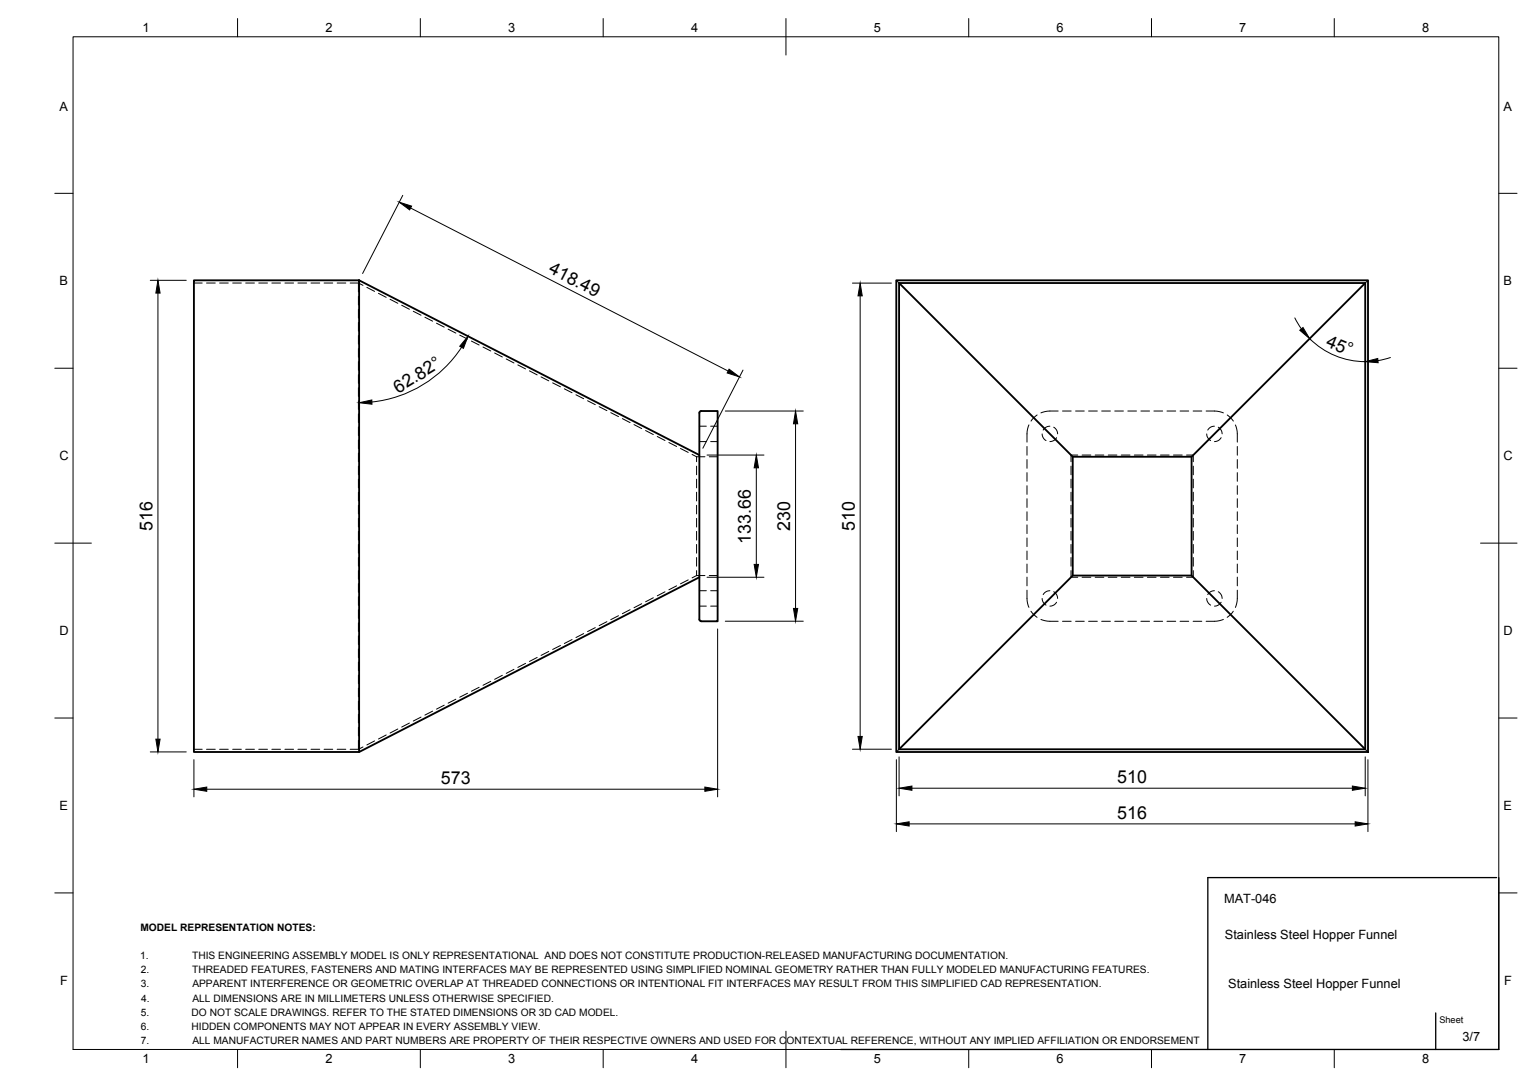
ISO-10303-21;
HEADER;
/* Generated by software containing ST-Developer
 * from STEP Tools, Inc. (www.steptools.com) 
 */

FILE_DESCRIPTION(
/* description */ ('STEP AP214'),
/* implementation_level */ '2;1');

FILE_NAME(
/* name */ 'Stainless Steel Hopper Funnel.step',
/* time_stamp */ '2026-11-14T22:16:48-08:00',
/* author */ (''),
/* organization */ (''),
/* preprocessor_version */ 'ST-DEVELOPER v20.2',
/* originating_system */ 'Autodesk Translation Framework v15.17.0.0',
/* authorisation */ '');

FILE_SCHEMA (('AUTOMOTIVE_DESIGN { 1 0 10303 214 3 1 1 }'));
ENDSEC;

DATA;
#10=MECHANICAL_DESIGN_GEOMETRIC_PRESENTATION_REPRESENTATION('',(#5472),#276462);
#5460=SHAPE_REPRESENTATION_RELATIONSHIP('SRR','None',#276488,#5466);
#5466=ADVANCED_BREP_SHAPE_REPRESENTATION('',(#5501),#276456);
#5472=STYLED_ITEM('',(#276527),#5501);
#5501=MANIFOLD_SOLID_BREP('Body1',#98697);
#5529=TOROIDAL_SURFACE('',#98859,23.,2.);
#5530=TOROIDAL_SURFACE('',#98866,23.,2.);
#5531=TOROIDAL_SURFACE('',#98868,23.,2.);
#5532=TOROIDAL_SURFACE('',#98874,23.,2.);
#6322=FACE_BOUND('',#13733,.T.);
#6323=FACE_BOUND('',#13751,.T.);
#6324=FACE_BOUND('',#13752,.T.);
#6325=FACE_BOUND('',#13753,.T.);
#6326=FACE_BOUND('',#13754,.T.);
#6327=FACE_BOUND('',#13755,.T.);
#6328=FACE_BOUND('',#13757,.T.);
#6329=FACE_BOUND('',#13758,.T.);
#6330=FACE_BOUND('',#13759,.T.);
#6331=FACE_BOUND('',#13760,.T.);
#6332=FACE_BOUND('',#13761,.T.);
#6446=PLANE('',#98816);
#6447=PLANE('',#98817);
#6448=PLANE('',#98818);
#6449=PLANE('',#98819);
#6450=PLANE('',#98820);
#6451=PLANE('',#98821);
#6452=PLANE('',#98822);
#6453=PLANE('',#98823);
#6454=PLANE('',#98824);
#6455=PLANE('',#98825);
#6456=PLANE('',#98826);
#6457=PLANE('',#98827);
#6458=PLANE('',#98828);
#6459=PLANE('',#98829);
#6460=PLANE('',#98830);
#6461=PLANE('',#98831);
#6462=PLANE('',#98832);
#6463=PLANE('',#98833);
#6464=PLANE('',#98834);
#6465=PLANE('',#98835);
#6466=PLANE('',#98836);
#6467=PLANE('',#98837);
#6468=PLANE('',#98842);
#6469=PLANE('',#98847);
#6470=PLANE('',#98848);
#6471=PLANE('',#98849);
#6472=PLANE('',#98850);
#7614=FACE_OUTER_BOUND('',#13724,.T.);
#7615=FACE_OUTER_BOUND('',#13725,.T.);
#7616=FACE_OUTER_BOUND('',#13726,.T.);
#7617=FACE_OUTER_BOUND('',#13727,.T.);
#7618=FACE_OUTER_BOUND('',#13728,.T.);
#7619=FACE_OUTER_BOUND('',#13729,.T.);
#7620=FACE_OUTER_BOUND('',#13730,.T.);
#7621=FACE_OUTER_BOUND('',#13731,.T.);
#7622=FACE_OUTER_BOUND('',#13732,.T.);
#7623=FACE_OUTER_BOUND('',#13734,.T.);
#7624=FACE_OUTER_BOUND('',#13735,.T.);
#7625=FACE_OUTER_BOUND('',#13736,.T.);
#7626=FACE_OUTER_BOUND('',#13737,.T.);
#7627=FACE_OUTER_BOUND('',#13738,.T.);
#7628=FACE_OUTER_BOUND('',#13739,.T.);
#7629=FACE_OUTER_BOUND('',#13740,.T.);
#7630=FACE_OUTER_BOUND('',#13741,.T.);
#7631=FACE_OUTER_BOUND('',#13742,.T.);
#7632=FACE_OUTER_BOUND('',#13743,.T.);
#7633=FACE_OUTER_BOUND('',#13744,.T.);
#7634=FACE_OUTER_BOUND('',#13745,.T.);
#7635=FACE_OUTER_BOUND('',#13746,.T.);
#7636=FACE_OUTER_BOUND('',#13747,.T.);
#7637=FACE_OUTER_BOUND('',#13748,.T.);
#7638=FACE_OUTER_BOUND('',#13749,.T.);
#7639=FACE_OUTER_BOUND('',#13750,.T.);
#7640=FACE_OUTER_BOUND('',#13756,.T.);
#7641=FACE_OUTER_BOUND('',#13762,.T.);
#7642=FACE_OUTER_BOUND('',#13763,.T.);
#7643=FACE_OUTER_BOUND('',#13764,.T.);
#7644=FACE_OUTER_BOUND('',#13765,.T.);
#7645=FACE_OUTER_BOUND('',#13766,.T.);
#7646=FACE_OUTER_BOUND('',#13767,.T.);
#7647=FACE_OUTER_BOUND('',#13768,.T.);
#7648=FACE_OUTER_BOUND('',#13769,.T.);
#7649=FACE_OUTER_BOUND('',#13770,.T.);
#7650=FACE_OUTER_BOUND('',#13771,.T.);
#7651=FACE_OUTER_BOUND('',#13772,.T.);
#7652=FACE_OUTER_BOUND('',#13773,.T.);
#7653=FACE_OUTER_BOUND('',#13774,.T.);
#7654=FACE_OUTER_BOUND('',#13775,.T.);
#7655=FACE_OUTER_BOUND('',#13776,.T.);
#7656=FACE_OUTER_BOUND('',#13777,.T.);
#13724=EDGE_LOOP('',(#60425,#60426,#60427,#60428));
#13725=EDGE_LOOP('',(#60429,#60430,#60431,#60432));
#13726=EDGE_LOOP('',(#60433,#60434,#60435,#60436));
#13727=EDGE_LOOP('',(#60437,#60438,#60439,#60440));
#13728=EDGE_LOOP('',(#60441,#60442,#60443,#60444));
#13729=EDGE_LOOP('',(#60445,#60446,#60447,#60448));
#13730=EDGE_LOOP('',(#60449,#60450,#60451,#60452));
#13731=EDGE_LOOP('',(#60453,#60454,#60455,#60456));
#13732=EDGE_LOOP('',(#60457,#60458,#60459,#60460));
#13733=EDGE_LOOP('',(#60461,#60462,#60463,#60464));
#13734=EDGE_LOOP('',(#60465,#60466,#60467,#60468));
#13735=EDGE_LOOP('',(#60469,#60470,#60471,#60472));
#13736=EDGE_LOOP('',(#60473,#60474,#60475,#60476));
#13737=EDGE_LOOP('',(#60477,#60478,#60479,#60480));
#13738=EDGE_LOOP('',(#60481,#60482,#60483,#60484));
#13739=EDGE_LOOP('',(#60485,#60486,#60487,#60488));
#13740=EDGE_LOOP('',(#60489,#60490,#60491,#60492));
#13741=EDGE_LOOP('',(#60493,#60494,#60495,#60496));
#13742=EDGE_LOOP('',(#60497,#60498,#60499,#60500));
#13743=EDGE_LOOP('',(#60501,#60502,#60503,#60504));
#13744=EDGE_LOOP('',(#60505,#60506,#60507,#60508));
#13745=EDGE_LOOP('',(#60509,#60510,#60511,#60512));
#13746=EDGE_LOOP('',(#60513,#60514,#60515,#60516));
#13747=EDGE_LOOP('',(#60517,#60518,#60519,#60520));
#13748=EDGE_LOOP('',(#60521,#60522,#60523,#60524));
#13749=EDGE_LOOP('',(#60525,#60526,#60527,#60528));
#13750=EDGE_LOOP('',(#60529,#60530,#60531,#60532,#60533,#60534,#60535,#60536));
#13751=EDGE_LOOP('',(#60537));
#13752=EDGE_LOOP('',(#60538));
#13753=EDGE_LOOP('',(#60539));
#13754=EDGE_LOOP('',(#60540));
#13755=EDGE_LOOP('',(#60541,#60542,#60543,#60544));
#13756=EDGE_LOOP('',(#60545,#60546,#60547,#60548,#60549,#60550,#60551,#60552));
#13757=EDGE_LOOP('',(#60553,#60554,#60555,#60556));
#13758=EDGE_LOOP('',(#60557));
#13759=EDGE_LOOP('',(#60558));
#13760=EDGE_LOOP('',(#60559));
#13761=EDGE_LOOP('',(#60560));
#13762=EDGE_LOOP('',(#60561,#60562,#60563,#60564));
#13763=EDGE_LOOP('',(#60565,#60566,#60567,#60568));
#13764=EDGE_LOOP('',(#60569,#60570,#60571,#60572));
#13765=EDGE_LOOP('',(#60573,#60574,#60575,#60576));
#13766=EDGE_LOOP('',(#60577,#60578,#60579,#60580));
#13767=EDGE_LOOP('',(#60581,#60582,#60583,#60584));
#13768=EDGE_LOOP('',(#60585,#60586,#60587,#60588));
#13769=EDGE_LOOP('',(#60589,#60590,#60591,#60592));
#13770=EDGE_LOOP('',(#60593,#60594,#60595,#60596));
#13771=EDGE_LOOP('',(#60597,#60598,#60599,#60600));
#13772=EDGE_LOOP('',(#60601,#60602,#60603,#60604));
#13773=EDGE_LOOP('',(#60605,#60606,#60607,#60608));
#13774=EDGE_LOOP('',(#60609,#60610,#60611,#60612));
#13775=EDGE_LOOP('',(#60613,#60614,#60615,#60616));
#13776=EDGE_LOOP('',(#60617,#60618,#60619,#60620));
#13777=EDGE_LOOP('',(#60621,#60622,#60623,#60624));
#19958=LINE('',#142648,#25185);
#19959=LINE('',#142654,#25186);
#19960=LINE('',#142660,#25187);
#19961=LINE('',#142666,#25188);
#19962=LINE('',#142671,#25189);
#19963=LINE('',#142673,#25190);
#19964=LINE('',#142675,#25191);
#19965=LINE('',#142676,#25192);
#19966=LINE('',#142679,#25193);
#19967=LINE('',#142681,#25194);
#19968=LINE('',#142682,#25195);
#19969=LINE('',#142685,#25196);
#19970=LINE('',#142687,#25197);
#19971=LINE('',#142688,#25198);
#19972=LINE('',#142690,#25199);
#19973=LINE('',#142691,#25200);
#19974=LINE('',#142695,#25201);
#19975=LINE('',#142697,#25202);
#19976=LINE('',#142699,#25203);
#19977=LINE('',#142700,#25204);
#19978=LINE('',#142703,#25205);
#19979=LINE('',#142705,#25206);
#19980=LINE('',#142706,#25207);
#19981=LINE('',#142709,#25208);
#19982=LINE('',#142710,#25209);
#19983=LINE('',#142713,#25210);
#19984=LINE('',#142714,#25211);
#19985=LINE('',#142716,#25212);
#19986=LINE('',#142719,#25213);
#19987=LINE('',#142721,#25214);
#19988=LINE('',#142722,#25215);
#19989=LINE('',#142725,#25216);
#19990=LINE('',#142726,#25217);
#19991=LINE('',#142729,#25218);
#19992=LINE('',#142730,#25219);
#19993=LINE('',#142732,#25220);
#19994=LINE('',#142735,#25221);
#19995=LINE('',#142737,#25222);
#19996=LINE('',#142738,#25223);
#19997=LINE('',#142741,#25224);
#19998=LINE('',#142742,#25225);
#19999=LINE('',#142745,#25226);
#20000=LINE('',#142746,#25227);
#20001=LINE('',#142748,#25228);
#20002=LINE('',#142751,#25229);
#20003=LINE('',#142753,#25230);
#20004=LINE('',#142754,#25231);
#20005=LINE('',#142757,#25232);
#20006=LINE('',#142758,#25233);
#20007=LINE('',#142761,#25234);
#20008=LINE('',#142762,#25235);
#20009=LINE('',#142764,#25236);
#20010=LINE('',#142768,#25237);
#20011=LINE('',#142772,#25238);
#20012=LINE('',#142776,#25239);
#20013=LINE('',#142780,#25240);
#20014=LINE('',#142785,#25241);
#20015=LINE('',#142789,#25242);
#20016=LINE('',#142793,#25243);
#20017=LINE('',#142797,#25244);
#20018=LINE('',#142801,#25245);
#20019=LINE('',#142803,#25246);
#20020=LINE('',#142804,#25247);
#20021=LINE('',#142807,#25248);
#20022=LINE('',#142809,#25249);
#20023=LINE('',#142810,#25250);
#20024=LINE('',#142813,#25251);
#20025=LINE('',#142815,#25252);
#20026=LINE('',#142816,#25253);
#20027=LINE('',#142819,#25254);
#20028=LINE('',#142821,#25255);
#20029=LINE('',#142822,#25256);
#25185=VECTOR('',#111681,8.4455);
#25186=VECTOR('',#111688,8.4455);
#25187=VECTOR('',#111695,8.4455);
#25188=VECTOR('',#111702,8.4455);
#25189=VECTOR('',#111707,1000.);
#25190=VECTOR('',#111708,1000.);
#25191=VECTOR('',#111709,1000.);
#25192=VECTOR('',#111710,1000.);
#25193=VECTOR('',#111713,1000.);
#25194=VECTOR('',#111714,1000.);
#25195=VECTOR('',#111715,1000.);
#25196=VECTOR('',#111718,1000.);
#25197=VECTOR('',#111719,1000.);
#25198=VECTOR('',#111720,1000.);
#25199=VECTOR('',#111723,1000.);
#25200=VECTOR('',#111724,1000.);
#25201=VECTOR('',#111727,1000.);
#25202=VECTOR('',#111728,1000.);
#25203=VECTOR('',#111729,1000.);
#25204=VECTOR('',#111730,1000.);
#25205=VECTOR('',#111733,1000.);
#25206=VECTOR('',#111734,1000.);
#25207=VECTOR('',#111735,1000.);
#25208=VECTOR('',#111738,1000.);
#25209=VECTOR('',#111739,1000.);
#25210=VECTOR('',#111742,1000.);
#25211=VECTOR('',#111743,1000.);
#25212=VECTOR('',#111746,1000.);
#25213=VECTOR('',#111749,1000.);
#25214=VECTOR('',#111750,1000.);
#25215=VECTOR('',#111751,1000.);
#25216=VECTOR('',#111754,1000.);
#25217=VECTOR('',#111755,1000.);
#25218=VECTOR('',#111758,1000.);
#25219=VECTOR('',#111759,1000.);
#25220=VECTOR('',#111762,1000.);
#25221=VECTOR('',#111765,1000.);
#25222=VECTOR('',#111766,1000.);
#25223=VECTOR('',#111767,1000.);
#25224=VECTOR('',#111770,1000.);
#25225=VECTOR('',#111771,1000.);
#25226=VECTOR('',#111774,1000.);
#25227=VECTOR('',#111775,1000.);
#25228=VECTOR('',#111778,1000.);
#25229=VECTOR('',#111781,1000.);
#25230=VECTOR('',#111782,1000.);
#25231=VECTOR('',#111783,1000.);
#25232=VECTOR('',#111786,1000.);
#25233=VECTOR('',#111787,1000.);
#25234=VECTOR('',#111790,1000.);
#25235=VECTOR('',#111791,1000.);
#25236=VECTOR('',#111794,1000.);
#25237=VECTOR('',#111797,1000.);
#25238=VECTOR('',#111800,1000.);
#25239=VECTOR('',#111803,1000.);
#25240=VECTOR('',#111806,1000.);
#25241=VECTOR('',#111811,1000.);
#25242=VECTOR('',#111814,1000.);
#25243=VECTOR('',#111817,1000.);
#25244=VECTOR('',#111820,1000.);
#25245=VECTOR('',#111825,1000.);
#25246=VECTOR('',#111826,1000.);
#25247=VECTOR('',#111827,1000.);
#25248=VECTOR('',#111830,1000.);
#25249=VECTOR('',#111831,1000.);
#25250=VECTOR('',#111832,1000.);
#25251=VECTOR('',#111835,1000.);
#25252=VECTOR('',#111836,1000.);
#25253=VECTOR('',#111837,1000.);
#25254=VECTOR('',#111840,1000.);
#25255=VECTOR('',#111841,1000.);
#25256=VECTOR('',#111842,1000.);
#30412=CIRCLE('',#98805,8.4455);
#30413=CIRCLE('',#98806,8.4455);
#30414=CIRCLE('',#98808,8.4455);
#30415=CIRCLE('',#98809,8.4455);
#30416=CIRCLE('',#98811,8.4455);
#30417=CIRCLE('',#98812,8.4455);
#30418=CIRCLE('',#98814,8.4455);
#30419=CIRCLE('',#98815,8.4455);
#30420=CIRCLE('',#98838,23.);
#30421=CIRCLE('',#98839,23.);
#30422=CIRCLE('',#98840,23.);
#30423=CIRCLE('',#98841,23.);
#30424=CIRCLE('',#98843,25.);
#30425=CIRCLE('',#98844,25.);
#30426=CIRCLE('',#98845,25.);
#30427=CIRCLE('',#98846,25.);
#30428=CIRCLE('',#98852,25.);
#30429=CIRCLE('',#98854,25.);
#30430=CIRCLE('',#98856,25.);
#30431=CIRCLE('',#98858,25.);
#30432=CIRCLE('',#98860,2.);
#30433=CIRCLE('',#98861,2.);
#30434=CIRCLE('',#98863,2.);
#30435=CIRCLE('',#98865,2.);
#30436=CIRCLE('',#98867,2.);
#30437=CIRCLE('',#98869,2.);
#30438=CIRCLE('',#98871,2.);
#30439=CIRCLE('',#98873,2.);
#36559=VERTEX_POINT('',#142645);
#36560=VERTEX_POINT('',#142647);
#36561=VERTEX_POINT('',#142651);
#36562=VERTEX_POINT('',#142653);
#36563=VERTEX_POINT('',#142657);
#36564=VERTEX_POINT('',#142659);
#36565=VERTEX_POINT('',#142663);
#36566=VERTEX_POINT('',#142665);
#36567=VERTEX_POINT('',#142669);
#36568=VERTEX_POINT('',#142670);
#36569=VERTEX_POINT('',#142672);
#36570=VERTEX_POINT('',#142674);
#36571=VERTEX_POINT('',#142678);
#36572=VERTEX_POINT('',#142680);
#36573=VERTEX_POINT('',#142684);
#36574=VERTEX_POINT('',#142686);
#36575=VERTEX_POINT('',#142693);
#36576=VERTEX_POINT('',#142694);
#36577=VERTEX_POINT('',#142696);
#36578=VERTEX_POINT('',#142698);
#36579=VERTEX_POINT('',#142702);
#36580=VERTEX_POINT('',#142704);
#36581=VERTEX_POINT('',#142708);
#36582=VERTEX_POINT('',#142712);
#36583=VERTEX_POINT('',#142718);
#36584=VERTEX_POINT('',#142720);
#36585=VERTEX_POINT('',#142724);
#36586=VERTEX_POINT('',#142728);
#36587=VERTEX_POINT('',#142734);
#36588=VERTEX_POINT('',#142736);
#36589=VERTEX_POINT('',#142740);
#36590=VERTEX_POINT('',#142744);
#36591=VERTEX_POINT('',#142750);
#36592=VERTEX_POINT('',#142752);
#36593=VERTEX_POINT('',#142756);
#36594=VERTEX_POINT('',#142760);
#36595=VERTEX_POINT('',#142766);
#36596=VERTEX_POINT('',#142767);
#36597=VERTEX_POINT('',#142769);
#36598=VERTEX_POINT('',#142771);
#36599=VERTEX_POINT('',#142773);
#36600=VERTEX_POINT('',#142775);
#36601=VERTEX_POINT('',#142777);
#36602=VERTEX_POINT('',#142779);
#36603=VERTEX_POINT('',#142783);
#36604=VERTEX_POINT('',#142784);
#36605=VERTEX_POINT('',#142786);
#36606=VERTEX_POINT('',#142788);
#36607=VERTEX_POINT('',#142790);
#36608=VERTEX_POINT('',#142792);
#36609=VERTEX_POINT('',#142794);
#36610=VERTEX_POINT('',#142796);
#36611=VERTEX_POINT('',#142800);
#36612=VERTEX_POINT('',#142802);
#36613=VERTEX_POINT('',#142806);
#36614=VERTEX_POINT('',#142808);
#36615=VERTEX_POINT('',#142812);
#36616=VERTEX_POINT('',#142814);
#36617=VERTEX_POINT('',#142818);
#36618=VERTEX_POINT('',#142820);
#45491=EDGE_CURVE('',#36559,#36559,#30412,.T.);
#45492=EDGE_CURVE('',#36559,#36560,#19958,.T.);
#45493=EDGE_CURVE('',#36560,#36560,#30413,.T.);
#45494=EDGE_CURVE('',#36561,#36561,#30414,.T.);
#45495=EDGE_CURVE('',#36561,#36562,#19959,.T.);
#45496=EDGE_CURVE('',#36562,#36562,#30415,.T.);
#45497=EDGE_CURVE('',#36563,#36563,#30416,.T.);
#45498=EDGE_CURVE('',#36563,#36564,#19960,.T.);
#45499=EDGE_CURVE('',#36564,#36564,#30417,.T.);
#45500=EDGE_CURVE('',#36565,#36565,#30418,.T.);
#45501=EDGE_CURVE('',#36565,#36566,#19961,.T.);
#45502=EDGE_CURVE('',#36566,#36566,#30419,.T.);
#45503=EDGE_CURVE('',#36567,#36568,#19962,.T.);
#45504=EDGE_CURVE('',#36569,#36567,#19963,.T.);
#45505=EDGE_CURVE('',#36569,#36570,#19964,.T.);
#45506=EDGE_CURVE('',#36570,#36568,#19965,.T.);
#45507=EDGE_CURVE('',#36571,#36567,#19966,.T.);
#45508=EDGE_CURVE('',#36572,#36571,#19967,.T.);
#45509=EDGE_CURVE('',#36572,#36569,#19968,.T.);
#45510=EDGE_CURVE('',#36573,#36571,#19969,.T.);
#45511=EDGE_CURVE('',#36574,#36573,#19970,.T.);
#45512=EDGE_CURVE('',#36574,#36572,#19971,.T.);
#45513=EDGE_CURVE('',#36568,#36573,#19972,.T.);
#45514=EDGE_CURVE('',#36570,#36574,#19973,.T.);
#45515=EDGE_CURVE('',#36575,#36576,#19974,.T.);
#45516=EDGE_CURVE('',#36577,#36575,#19975,.T.);
#45517=EDGE_CURVE('',#36578,#36577,#19976,.T.);
#45518=EDGE_CURVE('',#36576,#36578,#19977,.T.);
#45519=EDGE_CURVE('',#36579,#36574,#19978,.T.);
#45520=EDGE_CURVE('',#36580,#36570,#19979,.T.);
#45521=EDGE_CURVE('',#36579,#36580,#19980,.T.);
#45522=EDGE_CURVE('',#36581,#36569,#19981,.T.);
#45523=EDGE_CURVE('',#36580,#36581,#19982,.T.);
#45524=EDGE_CURVE('',#36582,#36572,#19983,.T.);
#45525=EDGE_CURVE('',#36582,#36579,#19984,.T.);
#45526=EDGE_CURVE('',#36581,#36582,#19985,.T.);
#45527=EDGE_CURVE('',#36583,#36576,#19986,.T.);
#45528=EDGE_CURVE('',#36584,#36583,#19987,.T.);
#45529=EDGE_CURVE('',#36584,#36575,#19988,.T.);
#45530=EDGE_CURVE('',#36585,#36584,#19989,.T.);
#45531=EDGE_CURVE('',#36585,#36577,#19990,.T.);
#45532=EDGE_CURVE('',#36586,#36585,#19991,.T.);
#45533=EDGE_CURVE('',#36586,#36578,#19992,.T.);
#45534=EDGE_CURVE('',#36583,#36586,#19993,.T.);
#45535=EDGE_CURVE('',#36587,#36586,#19994,.T.);
#45536=EDGE_CURVE('',#36587,#36588,#19995,.T.);
#45537=EDGE_CURVE('',#36588,#36583,#19996,.T.);
#45538=EDGE_CURVE('',#36588,#36589,#19997,.T.);
#45539=EDGE_CURVE('',#36589,#36584,#19998,.T.);
#45540=EDGE_CURVE('',#36590,#36585,#19999,.T.);
#45541=EDGE_CURVE('',#36590,#36587,#20000,.T.);
#45542=EDGE_CURVE('',#36589,#36590,#20001,.T.);
#45543=EDGE_CURVE('',#36591,#36587,#20002,.T.);
#45544=EDGE_CURVE('',#36591,#36592,#20003,.T.);
#45545=EDGE_CURVE('',#36592,#36588,#20004,.T.);
#45546=EDGE_CURVE('',#36592,#36593,#20005,.T.);
#45547=EDGE_CURVE('',#36593,#36589,#20006,.T.);
#45548=EDGE_CURVE('',#36593,#36594,#20007,.T.);
#45549=EDGE_CURVE('',#36594,#36590,#20008,.T.);
#45550=EDGE_CURVE('',#36594,#36591,#20009,.T.);
#45551=EDGE_CURVE('',#36595,#36596,#20010,.T.);
#45552=EDGE_CURVE('',#36596,#36597,#30420,.T.);
#45553=EDGE_CURVE('',#36597,#36598,#20011,.T.);
#45554=EDGE_CURVE('',#36598,#36599,#30421,.T.);
#45555=EDGE_CURVE('',#36599,#36600,#20012,.T.);
#45556=EDGE_CURVE('',#36600,#36601,#30422,.T.);
#45557=EDGE_CURVE('',#36601,#36602,#20013,.T.);
#45558=EDGE_CURVE('',#36602,#36595,#30423,.T.);
#45559=EDGE_CURVE('',#36603,#36604,#20014,.T.);
#45560=EDGE_CURVE('',#36604,#36605,#30424,.T.);
#45561=EDGE_CURVE('',#36605,#36606,#20015,.T.);
#45562=EDGE_CURVE('',#36606,#36607,#30425,.T.);
#45563=EDGE_CURVE('',#36607,#36608,#20016,.T.);
#45564=EDGE_CURVE('',#36608,#36609,#30426,.T.);
#45565=EDGE_CURVE('',#36609,#36610,#20017,.T.);
#45566=EDGE_CURVE('',#36610,#36603,#30427,.T.);
#45567=EDGE_CURVE('',#36603,#36611,#20018,.T.);
#45568=EDGE_CURVE('',#36611,#36612,#20019,.T.);
#45569=EDGE_CURVE('',#36612,#36604,#20020,.T.);
#45570=EDGE_CURVE('',#36605,#36613,#20021,.T.);
#45571=EDGE_CURVE('',#36613,#36614,#20022,.T.);
#45572=EDGE_CURVE('',#36614,#36606,#20023,.T.);
#45573=EDGE_CURVE('',#36607,#36615,#20024,.T.);
#45574=EDGE_CURVE('',#36615,#36616,#20025,.T.);
#45575=EDGE_CURVE('',#36616,#36608,#20026,.T.);
#45576=EDGE_CURVE('',#36609,#36617,#20027,.T.);
#45577=EDGE_CURVE('',#36617,#36618,#20028,.T.);
#45578=EDGE_CURVE('',#36618,#36610,#20029,.T.);
#45579=EDGE_CURVE('',#36612,#36613,#30428,.T.);
#45580=EDGE_CURVE('',#36618,#36611,#30429,.T.);
#45581=EDGE_CURVE('',#36616,#36617,#30430,.T.);
#45582=EDGE_CURVE('',#36614,#36615,#30431,.T.);
#45583=EDGE_CURVE('',#36615,#36600,#30432,.T.);
#45584=EDGE_CURVE('',#36601,#36614,#30433,.T.);
#45585=EDGE_CURVE('',#36602,#36613,#30434,.T.);
#45586=EDGE_CURVE('',#36616,#36599,#30435,.T.);
#45587=EDGE_CURVE('',#36595,#36612,#30436,.T.);
#45588=EDGE_CURVE('',#36617,#36598,#30437,.T.);
#45589=EDGE_CURVE('',#36596,#36611,#30438,.T.);
#45590=EDGE_CURVE('',#36618,#36597,#30439,.T.);
#60425=ORIENTED_EDGE('',*,*,#45491,.T.);
#60426=ORIENTED_EDGE('',*,*,#45492,.T.);
#60427=ORIENTED_EDGE('',*,*,#45493,.T.);
#60428=ORIENTED_EDGE('',*,*,#45492,.F.);
#60429=ORIENTED_EDGE('',*,*,#45494,.T.);
#60430=ORIENTED_EDGE('',*,*,#45495,.T.);
#60431=ORIENTED_EDGE('',*,*,#45496,.T.);
#60432=ORIENTED_EDGE('',*,*,#45495,.F.);
#60433=ORIENTED_EDGE('',*,*,#45497,.T.);
#60434=ORIENTED_EDGE('',*,*,#45498,.T.);
#60435=ORIENTED_EDGE('',*,*,#45499,.T.);
#60436=ORIENTED_EDGE('',*,*,#45498,.F.);
#60437=ORIENTED_EDGE('',*,*,#45500,.T.);
#60438=ORIENTED_EDGE('',*,*,#45501,.T.);
#60439=ORIENTED_EDGE('',*,*,#45502,.T.);
#60440=ORIENTED_EDGE('',*,*,#45501,.F.);
#60441=ORIENTED_EDGE('',*,*,#45503,.F.);
#60442=ORIENTED_EDGE('',*,*,#45504,.F.);
#60443=ORIENTED_EDGE('',*,*,#45505,.T.);
#60444=ORIENTED_EDGE('',*,*,#45506,.T.);
#60445=ORIENTED_EDGE('',*,*,#45507,.F.);
#60446=ORIENTED_EDGE('',*,*,#45508,.F.);
#60447=ORIENTED_EDGE('',*,*,#45509,.T.);
#60448=ORIENTED_EDGE('',*,*,#45504,.T.);
#60449=ORIENTED_EDGE('',*,*,#45510,.F.);
#60450=ORIENTED_EDGE('',*,*,#45511,.F.);
#60451=ORIENTED_EDGE('',*,*,#45512,.T.);
#60452=ORIENTED_EDGE('',*,*,#45508,.T.);
#60453=ORIENTED_EDGE('',*,*,#45513,.F.);
#60454=ORIENTED_EDGE('',*,*,#45506,.F.);
#60455=ORIENTED_EDGE('',*,*,#45514,.T.);
#60456=ORIENTED_EDGE('',*,*,#45511,.T.);
#60457=ORIENTED_EDGE('',*,*,#45503,.T.);
#60458=ORIENTED_EDGE('',*,*,#45513,.T.);
#60459=ORIENTED_EDGE('',*,*,#45510,.T.);
#60460=ORIENTED_EDGE('',*,*,#45507,.T.);
#60461=ORIENTED_EDGE('',*,*,#45515,.F.);
#60462=ORIENTED_EDGE('',*,*,#45516,.F.);
#60463=ORIENTED_EDGE('',*,*,#45517,.F.);
#60464=ORIENTED_EDGE('',*,*,#45518,.F.);
#60465=ORIENTED_EDGE('',*,*,#45519,.T.);
#60466=ORIENTED_EDGE('',*,*,#45514,.F.);
#60467=ORIENTED_EDGE('',*,*,#45520,.F.);
#60468=ORIENTED_EDGE('',*,*,#45521,.F.);
#60469=ORIENTED_EDGE('',*,*,#45520,.T.);
#60470=ORIENTED_EDGE('',*,*,#45505,.F.);
#60471=ORIENTED_EDGE('',*,*,#45522,.F.);
#60472=ORIENTED_EDGE('',*,*,#45523,.F.);
#60473=ORIENTED_EDGE('',*,*,#45524,.T.);
#60474=ORIENTED_EDGE('',*,*,#45512,.F.);
#60475=ORIENTED_EDGE('',*,*,#45519,.F.);
#60476=ORIENTED_EDGE('',*,*,#45525,.F.);
#60477=ORIENTED_EDGE('',*,*,#45522,.T.);
#60478=ORIENTED_EDGE('',*,*,#45509,.F.);
#60479=ORIENTED_EDGE('',*,*,#45524,.F.);
#60480=ORIENTED_EDGE('',*,*,#45526,.F.);
#60481=ORIENTED_EDGE('',*,*,#45515,.T.);
#60482=ORIENTED_EDGE('',*,*,#45527,.F.);
#60483=ORIENTED_EDGE('',*,*,#45528,.F.);
#60484=ORIENTED_EDGE('',*,*,#45529,.T.);
#60485=ORIENTED_EDGE('',*,*,#45516,.T.);
#60486=ORIENTED_EDGE('',*,*,#45529,.F.);
#60487=ORIENTED_EDGE('',*,*,#45530,.F.);
#60488=ORIENTED_EDGE('',*,*,#45531,.T.);
#60489=ORIENTED_EDGE('',*,*,#45517,.T.);
#60490=ORIENTED_EDGE('',*,*,#45531,.F.);
#60491=ORIENTED_EDGE('',*,*,#45532,.F.);
#60492=ORIENTED_EDGE('',*,*,#45533,.T.);
#60493=ORIENTED_EDGE('',*,*,#45518,.T.);
#60494=ORIENTED_EDGE('',*,*,#45533,.F.);
#60495=ORIENTED_EDGE('',*,*,#45534,.F.);
#60496=ORIENTED_EDGE('',*,*,#45527,.T.);
#60497=ORIENTED_EDGE('',*,*,#45535,.F.);
#60498=ORIENTED_EDGE('',*,*,#45536,.T.);
#60499=ORIENTED_EDGE('',*,*,#45537,.T.);
#60500=ORIENTED_EDGE('',*,*,#45534,.T.);
#60501=ORIENTED_EDGE('',*,*,#45537,.F.);
#60502=ORIENTED_EDGE('',*,*,#45538,.T.);
#60503=ORIENTED_EDGE('',*,*,#45539,.T.);
#60504=ORIENTED_EDGE('',*,*,#45528,.T.);
#60505=ORIENTED_EDGE('',*,*,#45540,.F.);
#60506=ORIENTED_EDGE('',*,*,#45541,.T.);
#60507=ORIENTED_EDGE('',*,*,#45535,.T.);
#60508=ORIENTED_EDGE('',*,*,#45532,.T.);
#60509=ORIENTED_EDGE('',*,*,#45539,.F.);
#60510=ORIENTED_EDGE('',*,*,#45542,.T.);
#60511=ORIENTED_EDGE('',*,*,#45540,.T.);
#60512=ORIENTED_EDGE('',*,*,#45530,.T.);
#60513=ORIENTED_EDGE('',*,*,#45543,.F.);
#60514=ORIENTED_EDGE('',*,*,#45544,.T.);
#60515=ORIENTED_EDGE('',*,*,#45545,.T.);
#60516=ORIENTED_EDGE('',*,*,#45536,.F.);
#60517=ORIENTED_EDGE('',*,*,#45545,.F.);
#60518=ORIENTED_EDGE('',*,*,#45546,.T.);
#60519=ORIENTED_EDGE('',*,*,#45547,.T.);
#60520=ORIENTED_EDGE('',*,*,#45538,.F.);
#60521=ORIENTED_EDGE('',*,*,#45547,.F.);
#60522=ORIENTED_EDGE('',*,*,#45548,.T.);
#60523=ORIENTED_EDGE('',*,*,#45549,.T.);
#60524=ORIENTED_EDGE('',*,*,#45542,.F.);
#60525=ORIENTED_EDGE('',*,*,#45549,.F.);
#60526=ORIENTED_EDGE('',*,*,#45550,.T.);
#60527=ORIENTED_EDGE('',*,*,#45543,.T.);
#60528=ORIENTED_EDGE('',*,*,#45541,.F.);
#60529=ORIENTED_EDGE('',*,*,#45551,.T.);
#60530=ORIENTED_EDGE('',*,*,#45552,.T.);
#60531=ORIENTED_EDGE('',*,*,#45553,.T.);
#60532=ORIENTED_EDGE('',*,*,#45554,.T.);
#60533=ORIENTED_EDGE('',*,*,#45555,.T.);
#60534=ORIENTED_EDGE('',*,*,#45556,.T.);
#60535=ORIENTED_EDGE('',*,*,#45557,.T.);
#60536=ORIENTED_EDGE('',*,*,#45558,.T.);
#60537=ORIENTED_EDGE('',*,*,#45491,.F.);
#60538=ORIENTED_EDGE('',*,*,#45494,.F.);
#60539=ORIENTED_EDGE('',*,*,#45497,.F.);
#60540=ORIENTED_EDGE('',*,*,#45500,.F.);
#60541=ORIENTED_EDGE('',*,*,#45526,.T.);
#60542=ORIENTED_EDGE('',*,*,#45525,.T.);
#60543=ORIENTED_EDGE('',*,*,#45521,.T.);
#60544=ORIENTED_EDGE('',*,*,#45523,.T.);
#60545=ORIENTED_EDGE('',*,*,#45559,.T.);
#60546=ORIENTED_EDGE('',*,*,#45560,.T.);
#60547=ORIENTED_EDGE('',*,*,#45561,.T.);
#60548=ORIENTED_EDGE('',*,*,#45562,.T.);
#60549=ORIENTED_EDGE('',*,*,#45563,.T.);
#60550=ORIENTED_EDGE('',*,*,#45564,.T.);
#60551=ORIENTED_EDGE('',*,*,#45565,.T.);
#60552=ORIENTED_EDGE('',*,*,#45566,.T.);
#60553=ORIENTED_EDGE('',*,*,#45548,.F.);
#60554=ORIENTED_EDGE('',*,*,#45546,.F.);
#60555=ORIENTED_EDGE('',*,*,#45544,.F.);
#60556=ORIENTED_EDGE('',*,*,#45550,.F.);
#60557=ORIENTED_EDGE('',*,*,#45493,.F.);
#60558=ORIENTED_EDGE('',*,*,#45496,.F.);
#60559=ORIENTED_EDGE('',*,*,#45499,.F.);
#60560=ORIENTED_EDGE('',*,*,#45502,.F.);
#60561=ORIENTED_EDGE('',*,*,#45567,.T.);
#60562=ORIENTED_EDGE('',*,*,#45568,.T.);
#60563=ORIENTED_EDGE('',*,*,#45569,.T.);
#60564=ORIENTED_EDGE('',*,*,#45559,.F.);
#60565=ORIENTED_EDGE('',*,*,#45570,.T.);
#60566=ORIENTED_EDGE('',*,*,#45571,.T.);
#60567=ORIENTED_EDGE('',*,*,#45572,.T.);
#60568=ORIENTED_EDGE('',*,*,#45561,.F.);
#60569=ORIENTED_EDGE('',*,*,#45573,.T.);
#60570=ORIENTED_EDGE('',*,*,#45574,.T.);
#60571=ORIENTED_EDGE('',*,*,#45575,.T.);
#60572=ORIENTED_EDGE('',*,*,#45563,.F.);
#60573=ORIENTED_EDGE('',*,*,#45576,.T.);
#60574=ORIENTED_EDGE('',*,*,#45577,.T.);
#60575=ORIENTED_EDGE('',*,*,#45578,.T.);
#60576=ORIENTED_EDGE('',*,*,#45565,.F.);
#60577=ORIENTED_EDGE('',*,*,#45569,.F.);
#60578=ORIENTED_EDGE('',*,*,#45579,.T.);
#60579=ORIENTED_EDGE('',*,*,#45570,.F.);
#60580=ORIENTED_EDGE('',*,*,#45560,.F.);
#60581=ORIENTED_EDGE('',*,*,#45578,.F.);
#60582=ORIENTED_EDGE('',*,*,#45580,.T.);
#60583=ORIENTED_EDGE('',*,*,#45567,.F.);
#60584=ORIENTED_EDGE('',*,*,#45566,.F.);
#60585=ORIENTED_EDGE('',*,*,#45575,.F.);
#60586=ORIENTED_EDGE('',*,*,#45581,.T.);
#60587=ORIENTED_EDGE('',*,*,#45576,.F.);
#60588=ORIENTED_EDGE('',*,*,#45564,.F.);
#60589=ORIENTED_EDGE('',*,*,#45572,.F.);
#60590=ORIENTED_EDGE('',*,*,#45582,.T.);
#60591=ORIENTED_EDGE('',*,*,#45573,.F.);
#60592=ORIENTED_EDGE('',*,*,#45562,.F.);
#60593=ORIENTED_EDGE('',*,*,#45583,.F.);
#60594=ORIENTED_EDGE('',*,*,#45582,.F.);
#60595=ORIENTED_EDGE('',*,*,#45584,.F.);
#60596=ORIENTED_EDGE('',*,*,#45556,.F.);
#60597=ORIENTED_EDGE('',*,*,#45584,.T.);
#60598=ORIENTED_EDGE('',*,*,#45571,.F.);
#60599=ORIENTED_EDGE('',*,*,#45585,.F.);
#60600=ORIENTED_EDGE('',*,*,#45557,.F.);
#60601=ORIENTED_EDGE('',*,*,#45583,.T.);
#60602=ORIENTED_EDGE('',*,*,#45555,.F.);
#60603=ORIENTED_EDGE('',*,*,#45586,.F.);
#60604=ORIENTED_EDGE('',*,*,#45574,.F.);
#60605=ORIENTED_EDGE('',*,*,#45585,.T.);
#60606=ORIENTED_EDGE('',*,*,#45579,.F.);
#60607=ORIENTED_EDGE('',*,*,#45587,.F.);
#60608=ORIENTED_EDGE('',*,*,#45558,.F.);
#60609=ORIENTED_EDGE('',*,*,#45586,.T.);
#60610=ORIENTED_EDGE('',*,*,#45554,.F.);
#60611=ORIENTED_EDGE('',*,*,#45588,.F.);
#60612=ORIENTED_EDGE('',*,*,#45581,.F.);
#60613=ORIENTED_EDGE('',*,*,#45587,.T.);
#60614=ORIENTED_EDGE('',*,*,#45568,.F.);
#60615=ORIENTED_EDGE('',*,*,#45589,.F.);
#60616=ORIENTED_EDGE('',*,*,#45551,.F.);
#60617=ORIENTED_EDGE('',*,*,#45588,.T.);
#60618=ORIENTED_EDGE('',*,*,#45553,.F.);
#60619=ORIENTED_EDGE('',*,*,#45590,.F.);
#60620=ORIENTED_EDGE('',*,*,#45577,.F.);
#60621=ORIENTED_EDGE('',*,*,#45589,.T.);
#60622=ORIENTED_EDGE('',*,*,#45580,.F.);
#60623=ORIENTED_EDGE('',*,*,#45590,.T.);
#60624=ORIENTED_EDGE('',*,*,#45552,.F.);
#90293=CYLINDRICAL_SURFACE('',#98804,8.4455);
#90294=CYLINDRICAL_SURFACE('',#98807,8.4455);
#90295=CYLINDRICAL_SURFACE('',#98810,8.4455);
#90296=CYLINDRICAL_SURFACE('',#98813,8.4455);
#90297=CYLINDRICAL_SURFACE('',#98851,25.);
#90298=CYLINDRICAL_SURFACE('',#98853,25.);
#90299=CYLINDRICAL_SURFACE('',#98855,25.);
#90300=CYLINDRICAL_SURFACE('',#98857,25.);
#90301=CYLINDRICAL_SURFACE('',#98862,2.);
#90302=CYLINDRICAL_SURFACE('',#98864,2.);
#90303=CYLINDRICAL_SURFACE('',#98870,2.);
#90304=CYLINDRICAL_SURFACE('',#98872,2.);
#92587=ADVANCED_FACE('',(#7614),#90293,.F.);
#92588=ADVANCED_FACE('',(#7615),#90294,.F.);
#92589=ADVANCED_FACE('',(#7616),#90295,.F.);
#92590=ADVANCED_FACE('',(#7617),#90296,.F.);
#92591=ADVANCED_FACE('',(#7618),#6446,.T.);
#92592=ADVANCED_FACE('',(#7619),#6447,.T.);
#92593=ADVANCED_FACE('',(#7620),#6448,.T.);
#92594=ADVANCED_FACE('',(#7621),#6449,.T.);
#92595=ADVANCED_FACE('',(#7622,#6322),#6450,.T.);
#92596=ADVANCED_FACE('',(#7623),#6451,.T.);
#92597=ADVANCED_FACE('',(#7624),#6452,.T.);
#92598=ADVANCED_FACE('',(#7625),#6453,.T.);
#92599=ADVANCED_FACE('',(#7626),#6454,.T.);
#92600=ADVANCED_FACE('',(#7627),#6455,.F.);
#92601=ADVANCED_FACE('',(#7628),#6456,.F.);
#92602=ADVANCED_FACE('',(#7629),#6457,.F.);
#92603=ADVANCED_FACE('',(#7630),#6458,.F.);
#92604=ADVANCED_FACE('',(#7631),#6459,.F.);
#92605=ADVANCED_FACE('',(#7632),#6460,.F.);
#92606=ADVANCED_FACE('',(#7633),#6461,.F.);
#92607=ADVANCED_FACE('',(#7634),#6462,.F.);
#92608=ADVANCED_FACE('',(#7635),#6463,.F.);
#92609=ADVANCED_FACE('',(#7636),#6464,.F.);
#92610=ADVANCED_FACE('',(#7637),#6465,.F.);
#92611=ADVANCED_FACE('',(#7638),#6466,.F.);
#92612=ADVANCED_FACE('',(#7639,#6323,#6324,#6325,#6326,#6327),#6467,.F.);
#92613=ADVANCED_FACE('',(#7640,#6328,#6329,#6330,#6331,#6332),#6468,.T.);
#92614=ADVANCED_FACE('',(#7641),#6469,.F.);
#92615=ADVANCED_FACE('',(#7642),#6470,.F.);
#92616=ADVANCED_FACE('',(#7643),#6471,.F.);
#92617=ADVANCED_FACE('',(#7644),#6472,.F.);
#92618=ADVANCED_FACE('',(#7645),#90297,.T.);
#92619=ADVANCED_FACE('',(#7646),#90298,.T.);
#92620=ADVANCED_FACE('',(#7647),#90299,.T.);
#92621=ADVANCED_FACE('',(#7648),#90300,.T.);
#92622=ADVANCED_FACE('',(#7649),#5529,.T.);
#92623=ADVANCED_FACE('',(#7650),#90301,.T.);
#92624=ADVANCED_FACE('',(#7651),#90302,.T.);
#92625=ADVANCED_FACE('',(#7652),#5530,.T.);
#92626=ADVANCED_FACE('',(#7653),#5531,.T.);
#92627=ADVANCED_FACE('',(#7654),#90303,.T.);
#92628=ADVANCED_FACE('',(#7655),#90304,.T.);
#92629=ADVANCED_FACE('',(#7656),#5532,.T.);
#98697=CLOSED_SHELL('',(#92587,#92588,#92589,#92590,#92591,#92592,#92593,
#92594,#92595,#92596,#92597,#92598,#92599,#92600,#92601,#92602,#92603,#92604,
#92605,#92606,#92607,#92608,#92609,#92610,#92611,#92612,#92613,#92614,#92615,
#92616,#92617,#92618,#92619,#92620,#92621,#92622,#92623,#92624,#92625,#92626,
#92627,#92628,#92629));
#98803=AXIS2_PLACEMENT_3D('',#142643,#111675,#111676);
#98804=AXIS2_PLACEMENT_3D('',#142644,#111677,#111678);
#98805=AXIS2_PLACEMENT_3D('',#142646,#111679,#111680);
#98806=AXIS2_PLACEMENT_3D('',#142649,#111682,#111683);
#98807=AXIS2_PLACEMENT_3D('',#142650,#111684,#111685);
#98808=AXIS2_PLACEMENT_3D('',#142652,#111686,#111687);
#98809=AXIS2_PLACEMENT_3D('',#142655,#111689,#111690);
#98810=AXIS2_PLACEMENT_3D('',#142656,#111691,#111692);
#98811=AXIS2_PLACEMENT_3D('',#142658,#111693,#111694);
#98812=AXIS2_PLACEMENT_3D('',#142661,#111696,#111697);
#98813=AXIS2_PLACEMENT_3D('',#142662,#111698,#111699);
#98814=AXIS2_PLACEMENT_3D('',#142664,#111700,#111701);
#98815=AXIS2_PLACEMENT_3D('',#142667,#111703,#111704);
#98816=AXIS2_PLACEMENT_3D('',#142668,#111705,#111706);
#98817=AXIS2_PLACEMENT_3D('',#142677,#111711,#111712);
#98818=AXIS2_PLACEMENT_3D('',#142683,#111716,#111717);
#98819=AXIS2_PLACEMENT_3D('',#142689,#111721,#111722);
#98820=AXIS2_PLACEMENT_3D('',#142692,#111725,#111726);
#98821=AXIS2_PLACEMENT_3D('',#142701,#111731,#111732);
#98822=AXIS2_PLACEMENT_3D('',#142707,#111736,#111737);
#98823=AXIS2_PLACEMENT_3D('',#142711,#111740,#111741);
#98824=AXIS2_PLACEMENT_3D('',#142715,#111744,#111745);
#98825=AXIS2_PLACEMENT_3D('',#142717,#111747,#111748);
#98826=AXIS2_PLACEMENT_3D('',#142723,#111752,#111753);
#98827=AXIS2_PLACEMENT_3D('',#142727,#111756,#111757);
#98828=AXIS2_PLACEMENT_3D('',#142731,#111760,#111761);
#98829=AXIS2_PLACEMENT_3D('',#142733,#111763,#111764);
#98830=AXIS2_PLACEMENT_3D('',#142739,#111768,#111769);
#98831=AXIS2_PLACEMENT_3D('',#142743,#111772,#111773);
#98832=AXIS2_PLACEMENT_3D('',#142747,#111776,#111777);
#98833=AXIS2_PLACEMENT_3D('',#142749,#111779,#111780);
#98834=AXIS2_PLACEMENT_3D('',#142755,#111784,#111785);
#98835=AXIS2_PLACEMENT_3D('',#142759,#111788,#111789);
#98836=AXIS2_PLACEMENT_3D('',#142763,#111792,#111793);
#98837=AXIS2_PLACEMENT_3D('',#142765,#111795,#111796);
#98838=AXIS2_PLACEMENT_3D('',#142770,#111798,#111799);
#98839=AXIS2_PLACEMENT_3D('',#142774,#111801,#111802);
#98840=AXIS2_PLACEMENT_3D('',#142778,#111804,#111805);
#98841=AXIS2_PLACEMENT_3D('',#142781,#111807,#111808);
#98842=AXIS2_PLACEMENT_3D('',#142782,#111809,#111810);
#98843=AXIS2_PLACEMENT_3D('',#142787,#111812,#111813);
#98844=AXIS2_PLACEMENT_3D('',#142791,#111815,#111816);
#98845=AXIS2_PLACEMENT_3D('',#142795,#111818,#111819);
#98846=AXIS2_PLACEMENT_3D('',#142798,#111821,#111822);
#98847=AXIS2_PLACEMENT_3D('',#142799,#111823,#111824);
#98848=AXIS2_PLACEMENT_3D('',#142805,#111828,#111829);
#98849=AXIS2_PLACEMENT_3D('',#142811,#111833,#111834);
#98850=AXIS2_PLACEMENT_3D('',#142817,#111838,#111839);
#98851=AXIS2_PLACEMENT_3D('',#142823,#111843,#111844);
#98852=AXIS2_PLACEMENT_3D('',#142824,#111845,#111846);
#98853=AXIS2_PLACEMENT_3D('',#142825,#111847,#111848);
#98854=AXIS2_PLACEMENT_3D('',#142826,#111849,#111850);
#98855=AXIS2_PLACEMENT_3D('',#142827,#111851,#111852);
#98856=AXIS2_PLACEMENT_3D('',#142828,#111853,#111854);
#98857=AXIS2_PLACEMENT_3D('',#142829,#111855,#111856);
#98858=AXIS2_PLACEMENT_3D('',#142830,#111857,#111858);
#98859=AXIS2_PLACEMENT_3D('',#142831,#111859,#111860);
#98860=AXIS2_PLACEMENT_3D('',#142832,#111861,#111862);
#98861=AXIS2_PLACEMENT_3D('',#142833,#111863,#111864);
#98862=AXIS2_PLACEMENT_3D('',#142834,#111865,#111866);
#98863=AXIS2_PLACEMENT_3D('',#142835,#111867,#111868);
#98864=AXIS2_PLACEMENT_3D('',#142836,#111869,#111870);
#98865=AXIS2_PLACEMENT_3D('',#142837,#111871,#111872);
#98866=AXIS2_PLACEMENT_3D('',#142838,#111873,#111874);
#98867=AXIS2_PLACEMENT_3D('',#142839,#111875,#111876);
#98868=AXIS2_PLACEMENT_3D('',#142840,#111877,#111878);
#98869=AXIS2_PLACEMENT_3D('',#142841,#111879,#111880);
#98870=AXIS2_PLACEMENT_3D('',#142842,#111881,#111882);
#98871=AXIS2_PLACEMENT_3D('',#142843,#111883,#111884);
#98872=AXIS2_PLACEMENT_3D('',#142844,#111885,#111886);
#98873=AXIS2_PLACEMENT_3D('',#142845,#111887,#111888);
#98874=AXIS2_PLACEMENT_3D('',#142846,#111889,#111890);
#111675=DIRECTION('axis',(0.,0.,1.));
#111676=DIRECTION('refdir',(1.,0.,0.));
#111677=DIRECTION('center_axis',(0.,-1.,0.));
#111678=DIRECTION('ref_axis',(0.,0.,-1.));
#111679=DIRECTION('center_axis',(0.,1.,0.));
#111680=DIRECTION('ref_axis',(0.,0.,-1.));
#111681=DIRECTION('',(0.,-1.,0.));
#111682=DIRECTION('center_axis',(0.,-1.,0.));
#111683=DIRECTION('ref_axis',(0.,0.,-1.));
#111684=DIRECTION('center_axis',(0.,-1.,0.));
#111685=DIRECTION('ref_axis',(0.,0.,-1.));
#111686=DIRECTION('center_axis',(0.,1.,0.));
#111687=DIRECTION('ref_axis',(0.,0.,-1.));
#111688=DIRECTION('',(0.,-1.,0.));
#111689=DIRECTION('center_axis',(0.,-1.,0.));
#111690=DIRECTION('ref_axis',(0.,0.,-1.));
#111691=DIRECTION('center_axis',(0.,-1.,0.));
#111692=DIRECTION('ref_axis',(0.,0.,-1.));
#111693=DIRECTION('center_axis',(0.,1.,0.));
#111694=DIRECTION('ref_axis',(0.,0.,-1.));
#111695=DIRECTION('',(0.,-1.,0.));
#111696=DIRECTION('center_axis',(0.,-1.,0.));
#111697=DIRECTION('ref_axis',(0.,0.,-1.));
#111698=DIRECTION('center_axis',(0.,-1.,0.));
#111699=DIRECTION('ref_axis',(0.,0.,-1.));
#111700=DIRECTION('center_axis',(0.,1.,0.));
#111701=DIRECTION('ref_axis',(0.,0.,-1.));
#111702=DIRECTION('',(0.,-1.,0.));
#111703=DIRECTION('center_axis',(0.,-1.,0.));
#111704=DIRECTION('ref_axis',(0.,0.,-1.));
#111705=DIRECTION('center_axis',(1.,0.,-2.17690789142188E-16));
#111706=DIRECTION('ref_axis',(-2.17690789142188E-16,0.,-1.));
#111707=DIRECTION('',(-2.17690789142188E-16,0.,-1.));
#111708=DIRECTION('',(0.,1.,0.));
#111709=DIRECTION('',(-2.17690789142188E-16,-1.23259516440783E-32,-1.));
#111710=DIRECTION('',(0.,1.,0.));
#111711=DIRECTION('center_axis',(0.,0.,1.));
#111712=DIRECTION('ref_axis',(1.,0.,0.));
#111713=DIRECTION('',(1.,0.,0.));
#111714=DIRECTION('',(0.,1.,0.));
#111715=DIRECTION('',(1.,0.,0.));
#111716=DIRECTION('center_axis',(-1.,0.,1.08845394571094E-16));
#111717=DIRECTION('ref_axis',(1.08845394571094E-16,0.,1.));
#111718=DIRECTION('',(1.08845394571094E-16,0.,1.));
#111719=DIRECTION('',(0.,1.,0.));
#111720=DIRECTION('',(1.08845394571094E-16,-6.16297582203916E-33,1.));
#111721=DIRECTION('center_axis',(0.,0.,-1.));
#111722=DIRECTION('ref_axis',(-1.,0.,0.));
#111723=DIRECTION('',(-1.,0.,0.));
#111724=DIRECTION('',(-1.,0.,0.));
#111725=DIRECTION('center_axis',(0.,1.,0.));
#111726=DIRECTION('ref_axis',(0.,0.,1.));
#111727=DIRECTION('',(-2.17690789142188E-16,0.,-1.));
#111728=DIRECTION('',(1.,0.,0.));
#111729=DIRECTION('',(1.08845394571094E-16,0.,1.));
#111730=DIRECTION('',(-1.,0.,0.));
#111731=DIRECTION('center_axis',(0.,-0.456804684992628,-0.889567018143538));
#111732=DIRECTION('ref_axis',(0.,0.889567018143538,-0.456804684992628));
#111733=DIRECTION('',(-0.415505315998661,0.809141931155286,-0.415505315998661));
#111734=DIRECTION('',(0.415505315998661,0.809141931155287,-0.415505315998661));
#111735=DIRECTION('',(1.,0.,0.));
#111736=DIRECTION('center_axis',(0.889567018143538,-0.456804684992628,-1.9365054617453E-16));
#111737=DIRECTION('ref_axis',(0.456804684992628,0.889567018143538,1.95408218286693E-33));
#111738=DIRECTION('',(0.415505315998661,0.809141931155287,0.415505315998661));
#111739=DIRECTION('',(2.17690789142188E-16,0.,1.));
#111740=DIRECTION('center_axis',(-0.889567018143538,-0.456804684992628,
9.68252730872648E-17));
#111741=DIRECTION('ref_axis',(0.456804684992628,-0.889567018143538,-8.78056366297357E-35));
#111742=DIRECTION('',(-0.415505315998661,0.809141931155287,0.415505315998661));
#111743=DIRECTION('',(-1.08845394571094E-16,0.,-1.));
#111744=DIRECTION('center_axis',(0.,-0.456804684992628,0.889567018143538));
#111745=DIRECTION('ref_axis',(0.,-0.889567018143538,-0.456804684992628));
#111746=DIRECTION('',(-1.,0.,0.));
#111747=DIRECTION('center_axis',(1.,0.,-2.17690789142188E-16));
#111748=DIRECTION('ref_axis',(-2.17690789142188E-16,0.,-1.));
#111749=DIRECTION('',(0.,1.,0.));
#111750=DIRECTION('',(-2.17690789142188E-16,0.,-1.));
#111751=DIRECTION('',(0.,1.,0.));
#111752=DIRECTION('center_axis',(0.,0.,1.));
#111753=DIRECTION('ref_axis',(1.,0.,0.));
#111754=DIRECTION('',(1.,0.,0.));
#111755=DIRECTION('',(0.,1.,0.));
#111756=DIRECTION('center_axis',(-1.,0.,1.08845394571094E-16));
#111757=DIRECTION('ref_axis',(1.08845394571094E-16,0.,1.));
#111758=DIRECTION('',(1.08845394571094E-16,0.,1.));
#111759=DIRECTION('',(0.,1.,0.));
#111760=DIRECTION('center_axis',(0.,0.,-1.));
#111761=DIRECTION('ref_axis',(-1.,0.,0.));
#111762=DIRECTION('',(-1.,0.,0.));
#111763=DIRECTION('center_axis',(0.,-0.456804684992628,-0.889567018143538));
#111764=DIRECTION('ref_axis',(0.,0.889567018143538,-0.456804684992628));
#111765=DIRECTION('',(-0.415505315998661,0.809141931155286,-0.415505315998661));
#111766=DIRECTION('',(1.,0.,0.));
#111767=DIRECTION('',(0.41550531599866,0.809141931155286,-0.415505315998661));
#111768=DIRECTION('center_axis',(0.889567018143538,-0.456804684992628,-1.9365054617453E-16));
#111769=DIRECTION('ref_axis',(0.456804684992628,0.889567018143538,1.95408218286693E-33));
#111770=DIRECTION('',(0.,0.,1.));
#111771=DIRECTION('',(0.415505315998661,0.809141931155286,0.415505315998661));
#111772=DIRECTION('center_axis',(-0.889567018143538,-0.456804684992628,
9.68252730872648E-17));
#111773=DIRECTION('ref_axis',(0.456804684992628,-0.889567018143538,-8.78056366297357E-35));
#111774=DIRECTION('',(-0.415505315998661,0.809141931155287,0.415505315998661));
#111775=DIRECTION('',(2.1350442781253E-16,0.,-1.));
#111776=DIRECTION('center_axis',(0.,-0.456804684992628,0.889567018143538));
#111777=DIRECTION('ref_axis',(0.,-0.889567018143538,-0.456804684992628));
#111778=DIRECTION('',(-1.,0.,0.));
#111779=DIRECTION('center_axis',(0.,0.,-1.));
#111780=DIRECTION('ref_axis',(-1.,0.,0.));
#111781=DIRECTION('',(0.,1.,0.));
#111782=DIRECTION('',(1.,0.,0.));
#111783=DIRECTION('',(0.,1.,0.));
#111784=DIRECTION('center_axis',(1.,0.,0.));
#111785=DIRECTION('ref_axis',(0.,0.,-1.));
#111786=DIRECTION('',(0.,0.,1.));
#111787=DIRECTION('',(0.,1.,0.));
#111788=DIRECTION('center_axis',(0.,0.,1.));
#111789=DIRECTION('ref_axis',(1.,0.,0.));
#111790=DIRECTION('',(-1.,0.,0.));
#111791=DIRECTION('',(0.,1.,0.));
#111792=DIRECTION('center_axis',(-1.,0.,-2.1350442781253E-16));
#111793=DIRECTION('ref_axis',(-2.1350442781253E-16,0.,1.));
#111794=DIRECTION('',(0.,0.,-1.));
#111795=DIRECTION('center_axis',(0.,-1.,0.));
#111796=DIRECTION('ref_axis',(0.,0.,-1.));
#111797=DIRECTION('',(0.,0.,-1.));
#111798=DIRECTION('center_axis',(0.,1.,0.));
#111799=DIRECTION('ref_axis',(0.,0.,-1.));
#111800=DIRECTION('',(-1.,0.,0.));
#111801=DIRECTION('center_axis',(0.,1.,0.));
#111802=DIRECTION('ref_axis',(0.,0.,-1.));
#111803=DIRECTION('',(0.,0.,1.));
#111804=DIRECTION('center_axis',(0.,1.,0.));
#111805=DIRECTION('ref_axis',(0.,0.,-1.));
#111806=DIRECTION('',(1.,0.,0.));
#111807=DIRECTION('center_axis',(0.,1.,0.));
#111808=DIRECTION('ref_axis',(0.,0.,-1.));
#111809=DIRECTION('center_axis',(0.,-1.,0.));
#111810=DIRECTION('ref_axis',(0.,0.,-1.));
#111811=DIRECTION('',(0.,0.,1.));
#111812=DIRECTION('center_axis',(0.,-1.,0.));
#111813=DIRECTION('ref_axis',(0.,0.,-1.));
#111814=DIRECTION('',(-1.,0.,0.));
#111815=DIRECTION('center_axis',(0.,-1.,0.));
#111816=DIRECTION('ref_axis',(0.,0.,-1.));
#111817=DIRECTION('',(0.,0.,-1.));
#111818=DIRECTION('center_axis',(0.,-1.,0.));
#111819=DIRECTION('ref_axis',(0.,0.,-1.));
#111820=DIRECTION('',(1.,0.,0.));
#111821=DIRECTION('center_axis',(0.,-1.,0.));
#111822=DIRECTION('ref_axis',(0.,0.,-1.));
#111823=DIRECTION('center_axis',(-1.,0.,0.));
#111824=DIRECTION('ref_axis',(0.,0.,1.));
#111825=DIRECTION('',(0.,1.,0.));
#111826=DIRECTION('',(0.,0.,1.));
#111827=DIRECTION('',(0.,-1.,0.));
#111828=DIRECTION('center_axis',(0.,0.,-1.));
#111829=DIRECTION('ref_axis',(-1.,0.,0.));
#111830=DIRECTION('',(0.,1.,0.));
#111831=DIRECTION('',(-1.,0.,0.));
#111832=DIRECTION('',(0.,-1.,0.));
#111833=DIRECTION('center_axis',(1.,0.,0.));
#111834=DIRECTION('ref_axis',(0.,0.,-1.));
#111835=DIRECTION('',(0.,1.,0.));
#111836=DIRECTION('',(0.,0.,-1.));
#111837=DIRECTION('',(0.,-1.,0.));
#111838=DIRECTION('center_axis',(0.,0.,1.));
#111839=DIRECTION('ref_axis',(1.,0.,0.));
#111840=DIRECTION('',(0.,1.,0.));
#111841=DIRECTION('',(1.,0.,0.));
#111842=DIRECTION('',(0.,-1.,0.));
#111843=DIRECTION('center_axis',(0.,1.,0.));
#111844=DIRECTION('ref_axis',(0.,0.,1.));
#111845=DIRECTION('center_axis',(0.,-1.,0.));
#111846=DIRECTION('ref_axis',(0.,0.,-1.));
#111847=DIRECTION('center_axis',(0.,1.,0.));
#111848=DIRECTION('ref_axis',(0.,0.,1.));
#111849=DIRECTION('center_axis',(0.,-1.,0.));
#111850=DIRECTION('ref_axis',(0.,0.,-1.));
#111851=DIRECTION('center_axis',(0.,1.,0.));
#111852=DIRECTION('ref_axis',(0.,0.,1.));
#111853=DIRECTION('center_axis',(0.,-1.,0.));
#111854=DIRECTION('ref_axis',(0.,0.,-1.));
#111855=DIRECTION('center_axis',(0.,1.,0.));
#111856=DIRECTION('ref_axis',(0.,0.,1.));
#111857=DIRECTION('center_axis',(0.,-1.,0.));
#111858=DIRECTION('ref_axis',(0.,0.,-1.));
#111859=DIRECTION('center_axis',(0.,-1.,0.));
#111860=DIRECTION('ref_axis',(0.,0.,-1.));
#111861=DIRECTION('center_axis',(0.,0.,-1.));
#111862=DIRECTION('ref_axis',(-1.,0.,0.));
#111863=DIRECTION('center_axis',(1.,0.,0.));
#111864=DIRECTION('ref_axis',(0.,0.,-1.));
#111865=DIRECTION('center_axis',(-1.,0.,0.));
#111866=DIRECTION('ref_axis',(0.,0.,1.));
#111867=DIRECTION('center_axis',(1.,0.,0.));
#111868=DIRECTION('ref_axis',(0.,0.,-1.));
#111869=DIRECTION('center_axis',(0.,0.,-1.));
#111870=DIRECTION('ref_axis',(-1.,0.,0.));
#111871=DIRECTION('center_axis',(0.,0.,-1.));
#111872=DIRECTION('ref_axis',(-1.,0.,0.));
#111873=DIRECTION('center_axis',(0.,-1.,0.));
#111874=DIRECTION('ref_axis',(0.,0.,-1.));
#111875=DIRECTION('center_axis',(0.,0.,-1.));
#111876=DIRECTION('ref_axis',(-1.,0.,0.));
#111877=DIRECTION('center_axis',(0.,-1.,0.));
#111878=DIRECTION('ref_axis',(0.,0.,-1.));
#111879=DIRECTION('center_axis',(1.,0.,0.));
#111880=DIRECTION('ref_axis',(0.,0.,-1.));
#111881=DIRECTION('center_axis',(0.,0.,1.));
#111882=DIRECTION('ref_axis',(1.,0.,0.));
#111883=DIRECTION('center_axis',(0.,0.,-1.));
#111884=DIRECTION('ref_axis',(-1.,0.,0.));
#111885=DIRECTION('center_axis',(1.,0.,0.));
#111886=DIRECTION('ref_axis',(0.,0.,-1.));
#111887=DIRECTION('center_axis',(1.,0.,0.));
#111888=DIRECTION('ref_axis',(0.,0.,-1.));
#111889=DIRECTION('center_axis',(0.,-1.,0.));
#111890=DIRECTION('ref_axis',(0.,0.,-1.));
#142643=CARTESIAN_POINT('',(0.,0.,0.));
#142644=CARTESIAN_POINT('Origin',(90.,-529.112518717956,90.));
#142645=CARTESIAN_POINT('',(90.,-553.,98.4455));
#142646=CARTESIAN_POINT('Origin',(90.,-553.,90.));
#142647=CARTESIAN_POINT('',(90.,-573.,98.4455));
#142648=CARTESIAN_POINT('',(90.,-529.112518717956,98.4455));
#142649=CARTESIAN_POINT('Origin',(90.,-573.,90.));
#142650=CARTESIAN_POINT('Origin',(-90.,-529.112518717956,90.));
#142651=CARTESIAN_POINT('',(-90.,-553.,98.4455));
#142652=CARTESIAN_POINT('Origin',(-90.,-553.,90.));
#142653=CARTESIAN_POINT('',(-90.,-573.,98.4455));
#142654=CARTESIAN_POINT('',(-90.,-529.112518717956,98.4455));
#142655=CARTESIAN_POINT('Origin',(-90.,-573.,90.));
#142656=CARTESIAN_POINT('Origin',(-90.,-529.112518717956,-90.0000000000001));
#142657=CARTESIAN_POINT('',(-90.,-553.,-81.5545));
#142658=CARTESIAN_POINT('Origin',(-90.,-553.,-90.0000000000001));
#142659=CARTESIAN_POINT('',(-90.,-573.,-81.5545));
#142660=CARTESIAN_POINT('',(-90.,-529.112518717956,-81.5545));
#142661=CARTESIAN_POINT('Origin',(-90.,-573.,-90.0000000000001));
#142662=CARTESIAN_POINT('Origin',(90.,-529.112518717956,-90.));
#142663=CARTESIAN_POINT('',(90.,-553.,-81.5545));
#142664=CARTESIAN_POINT('Origin',(90.,-553.,-90.));
#142665=CARTESIAN_POINT('',(90.,-573.,-81.5545));
#142666=CARTESIAN_POINT('',(90.,-529.112518717956,-81.5545));
#142667=CARTESIAN_POINT('Origin',(90.,-573.,-90.));
#142668=CARTESIAN_POINT('Origin',(258.,-180.,-255.));
#142669=CARTESIAN_POINT('',(258.,0.,258.));
#142670=CARTESIAN_POINT('',(258.,0.,-258.));
#142671=CARTESIAN_POINT('',(258.,0.,-5.61642235986844E-14));
#142672=CARTESIAN_POINT('',(258.,-180.725252950448,258.));
#142673=CARTESIAN_POINT('',(258.,-180.,258.));
#142674=CARTESIAN_POINT('',(258.,-180.725252950448,-258.));
#142675=CARTESIAN_POINT('',(258.,-180.725252950448,-255.));
#142676=CARTESIAN_POINT('',(258.,-180.,-258.));
#142677=CARTESIAN_POINT('Origin',(-255.,-180.,258.));
#142678=CARTESIAN_POINT('',(-258.,0.,258.));
#142679=CARTESIAN_POINT('',(0.,0.,258.));
#142680=CARTESIAN_POINT('',(-258.,-180.725252950448,258.));
#142681=CARTESIAN_POINT('',(-258.,-180.,258.));
#142682=CARTESIAN_POINT('',(-255.,-180.725252950448,258.));
#142683=CARTESIAN_POINT('Origin',(-258.,-180.,-255.));
#142684=CARTESIAN_POINT('',(-258.,0.,-258.));
#142685=CARTESIAN_POINT('',(-258.,0.,2.80821117993422E-14));
#142686=CARTESIAN_POINT('',(-258.,-180.725252950448,-258.));
#142687=CARTESIAN_POINT('',(-258.,-180.,-258.));
#142688=CARTESIAN_POINT('',(-258.,-180.725252950448,-255.));
#142689=CARTESIAN_POINT('Origin',(-255.,-180.,-258.));
#142690=CARTESIAN_POINT('',(0.,0.,-258.));
#142691=CARTESIAN_POINT('',(-255.,-180.725252950448,-258.));
#142692=CARTESIAN_POINT('Origin',(0.,0.,0.));
#142693=CARTESIAN_POINT('',(255.,0.,255.));
#142694=CARTESIAN_POINT('',(255.,0.,-255.));
#142695=CARTESIAN_POINT('',(255.,0.,-255.));
#142696=CARTESIAN_POINT('',(-255.,0.,255.));
#142697=CARTESIAN_POINT('',(-255.,0.,255.));
#142698=CARTESIAN_POINT('',(-255.,0.,-255.));
#142699=CARTESIAN_POINT('',(-255.,0.,-255.));
#142700=CARTESIAN_POINT('',(-255.,0.,-255.));
#142701=CARTESIAN_POINT('Origin',(0.,-142.552494979833,-277.602227065991));
#142702=CARTESIAN_POINT('',(-66.83188665023,-553.,-66.8318866502301));
#142703=CARTESIAN_POINT('',(-229.675682842738,-235.88313373038,-229.675682842738));
#142704=CARTESIAN_POINT('',(66.8318866502301,-553.,-66.8318866502301));
#142705=CARTESIAN_POINT('',(229.675682842738,-235.883133730379,-229.675682842738));
#142706=CARTESIAN_POINT('',(0.,-553.,-66.8318866502301));
#142707=CARTESIAN_POINT('Origin',(277.602227065991,-142.552494979833,-6.04314478776244E-14));
#142708=CARTESIAN_POINT('',(66.8318866502301,-553.,66.8318866502301));
#142709=CARTESIAN_POINT('',(229.675682842738,-235.88313373038,229.675682842738));
#142710=CARTESIAN_POINT('',(66.8318866502301,-553.,-1.45486861447498E-14));
#142711=CARTESIAN_POINT('Origin',(-277.602227065991,-142.552494979833,3.02157239388122E-14));
#142712=CARTESIAN_POINT('',(-66.83188665023,-553.,66.8318866502301));
#142713=CARTESIAN_POINT('',(-229.675682842738,-235.883133730379,229.675682842738));
#142714=CARTESIAN_POINT('',(-66.83188665023,-553.,7.2743430723749E-15));
#142715=CARTESIAN_POINT('Origin',(0.,-142.552494979833,277.602227065991));
#142716=CARTESIAN_POINT('',(0.,-553.,66.8318866502301));
#142717=CARTESIAN_POINT('Origin',(255.,-180.,-255.));
#142718=CARTESIAN_POINT('',(255.,-180.,-255.));
#142719=CARTESIAN_POINT('',(255.,-180.,-255.));
#142720=CARTESIAN_POINT('',(255.,-180.,255.));
#142721=CARTESIAN_POINT('',(255.,-180.,-255.));
#142722=CARTESIAN_POINT('',(255.,-180.,255.));
#142723=CARTESIAN_POINT('Origin',(-255.,-180.,255.));
#142724=CARTESIAN_POINT('',(-255.,-180.,255.));
#142725=CARTESIAN_POINT('',(-255.,-180.,255.));
#142726=CARTESIAN_POINT('',(-255.,-180.,255.));
#142727=CARTESIAN_POINT('Origin',(-255.,-180.,-255.));
#142728=CARTESIAN_POINT('',(-255.,-180.,-255.));
#142729=CARTESIAN_POINT('',(-255.,-180.,-255.));
#142730=CARTESIAN_POINT('',(-255.,-180.,-255.));
#142731=CARTESIAN_POINT('Origin',(-255.,-180.,-255.));
#142732=CARTESIAN_POINT('',(-255.,-180.,-255.));
#142733=CARTESIAN_POINT('Origin',(0.,-141.182080924855,-274.933526011561));
#142734=CARTESIAN_POINT('',(-65.,-550.,-65.));
#142735=CARTESIAN_POINT('',(-65.,-550.,-65.));
#142736=CARTESIAN_POINT('',(65.,-550.,-65.));
#142737=CARTESIAN_POINT('',(65.,-550.,-65.));
#142738=CARTESIAN_POINT('',(65.,-550.,-65.));
#142739=CARTESIAN_POINT('Origin',(274.933526011561,-141.182080924855,-5.98504962391008E-14));
#142740=CARTESIAN_POINT('',(65.,-550.,65.));
#142741=CARTESIAN_POINT('',(65.,-550.,-65.));
#142742=CARTESIAN_POINT('',(65.,-550.,65.));
#142743=CARTESIAN_POINT('Origin',(-274.933526011561,-141.182080924855,2.99252481195504E-14));
#142744=CARTESIAN_POINT('',(-65.,-550.,65.));
#142745=CARTESIAN_POINT('',(-65.,-550.,65.));
#142746=CARTESIAN_POINT('',(-65.,-550.,-65.));
#142747=CARTESIAN_POINT('Origin',(0.,-141.182080924856,274.933526011561));
#142748=CARTESIAN_POINT('',(65.,-550.,65.));
#142749=CARTESIAN_POINT('Origin',(65.,-580.,-65.));
#142750=CARTESIAN_POINT('',(-64.9999999999999,-573.,-65.));
#142751=CARTESIAN_POINT('',(-65.,-580.,-65.));
#142752=CARTESIAN_POINT('',(65.,-573.,-65.));
#142753=CARTESIAN_POINT('',(-64.9999999999999,-573.,-65.));
#142754=CARTESIAN_POINT('',(65.,-580.,-65.));
#142755=CARTESIAN_POINT('Origin',(65.,-580.,65.));
#142756=CARTESIAN_POINT('',(65.,-573.,65.));
#142757=CARTESIAN_POINT('',(65.,-573.,65.));
#142758=CARTESIAN_POINT('',(65.,-580.,65.));
#142759=CARTESIAN_POINT('Origin',(-65.,-580.,65.));
#142760=CARTESIAN_POINT('',(-64.9999999999999,-573.,65.));
#142761=CARTESIAN_POINT('',(-64.9999999999999,-573.,65.));
#142762=CARTESIAN_POINT('',(-65.,-580.,65.));
#142763=CARTESIAN_POINT('Origin',(-65.,-580.,-65.));
#142764=CARTESIAN_POINT('',(-64.9999999999999,-573.,65.));
#142765=CARTESIAN_POINT('Origin',(0.,-553.,0.));
#142766=CARTESIAN_POINT('',(113.,-553.,90.));
#142767=CARTESIAN_POINT('',(113.,-553.,-90.));
#142768=CARTESIAN_POINT('',(113.,-553.,0.));
#142769=CARTESIAN_POINT('',(90.,-553.,-113.));
#142770=CARTESIAN_POINT('Origin',(90.,-553.,-90.));
#142771=CARTESIAN_POINT('',(-90.0000000000001,-553.,-113.));
#142772=CARTESIAN_POINT('',(0.,-553.,-113.));
#142773=CARTESIAN_POINT('',(-113.,-553.,-90.));
#142774=CARTESIAN_POINT('Origin',(-90.0000000000001,-553.,-90.));
#142775=CARTESIAN_POINT('',(-113.,-553.,90.));
#142776=CARTESIAN_POINT('',(-113.,-553.,0.));
#142777=CARTESIAN_POINT('',(-90.0000000000001,-553.,113.));
#142778=CARTESIAN_POINT('Origin',(-90.0000000000001,-553.,90.));
#142779=CARTESIAN_POINT('',(90.,-553.,113.));
#142780=CARTESIAN_POINT('',(0.,-553.,113.));
#142781=CARTESIAN_POINT('Origin',(90.,-553.,90.));
#142782=CARTESIAN_POINT('Origin',(0.,-573.,0.));
#142783=CARTESIAN_POINT('',(115.,-573.,-90.));
#142784=CARTESIAN_POINT('',(115.,-573.,90.));
#142785=CARTESIAN_POINT('',(115.,-573.,115.));
#142786=CARTESIAN_POINT('',(90.,-573.,115.));
#142787=CARTESIAN_POINT('Origin',(90.,-573.,90.));
#142788=CARTESIAN_POINT('',(-90.0000000000001,-573.,115.));
#142789=CARTESIAN_POINT('',(-115.,-573.,115.));
#142790=CARTESIAN_POINT('',(-115.,-573.,90.));
#142791=CARTESIAN_POINT('Origin',(-90.0000000000001,-573.,90.));
#142792=CARTESIAN_POINT('',(-115.,-573.,-90.));
#142793=CARTESIAN_POINT('',(-115.,-573.,115.));
#142794=CARTESIAN_POINT('',(-90.0000000000001,-573.,-115.));
#142795=CARTESIAN_POINT('Origin',(-90.0000000000001,-573.,-90.));
#142796=CARTESIAN_POINT('',(90.,-573.,-115.));
#142797=CARTESIAN_POINT('',(-115.,-573.,-115.));
#142798=CARTESIAN_POINT('Origin',(90.,-573.,-90.));
#142799=CARTESIAN_POINT('Origin',(115.,-573.,115.));
#142800=CARTESIAN_POINT('',(115.,-555.,-90.));
#142801=CARTESIAN_POINT('',(115.,-573.,-90.));
#142802=CARTESIAN_POINT('',(115.,-555.,90.));
#142803=CARTESIAN_POINT('',(115.,-555.,115.));
#142804=CARTESIAN_POINT('',(115.,-573.,90.));
#142805=CARTESIAN_POINT('Origin',(-115.,-573.,115.));
#142806=CARTESIAN_POINT('',(90.,-555.,115.));
#142807=CARTESIAN_POINT('',(90.,-573.,115.));
#142808=CARTESIAN_POINT('',(-90.0000000000001,-555.,115.));
#142809=CARTESIAN_POINT('',(-115.,-555.,115.));
#142810=CARTESIAN_POINT('',(-90.0000000000001,-573.,115.));
#142811=CARTESIAN_POINT('Origin',(-115.,-573.,115.));
#142812=CARTESIAN_POINT('',(-115.,-555.,90.));
#142813=CARTESIAN_POINT('',(-115.,-573.,90.));
#142814=CARTESIAN_POINT('',(-115.,-555.,-90.));
#142815=CARTESIAN_POINT('',(-115.,-555.,115.));
#142816=CARTESIAN_POINT('',(-115.,-573.,-90.));
#142817=CARTESIAN_POINT('Origin',(-115.,-573.,-115.));
#142818=CARTESIAN_POINT('',(-90.0000000000001,-555.,-115.));
#142819=CARTESIAN_POINT('',(-90.0000000000001,-573.,-115.));
#142820=CARTESIAN_POINT('',(90.,-555.,-115.));
#142821=CARTESIAN_POINT('',(-115.,-555.,-115.));
#142822=CARTESIAN_POINT('',(90.,-573.,-115.));
#142823=CARTESIAN_POINT('Origin',(90.,-573.,90.));
#142824=CARTESIAN_POINT('Origin',(90.,-555.,90.));
#142825=CARTESIAN_POINT('Origin',(90.,-573.,-90.));
#142826=CARTESIAN_POINT('Origin',(90.,-555.,-90.));
#142827=CARTESIAN_POINT('Origin',(-90.0000000000001,-573.,-90.));
#142828=CARTESIAN_POINT('Origin',(-90.0000000000001,-555.,-90.));
#142829=CARTESIAN_POINT('Origin',(-90.0000000000001,-573.,90.));
#142830=CARTESIAN_POINT('Origin',(-90.0000000000001,-555.,90.));
#142831=CARTESIAN_POINT('Origin',(-90.0000000000001,-555.,90.));
#142832=CARTESIAN_POINT('Origin',(-113.,-555.,90.));
#142833=CARTESIAN_POINT('Origin',(-90.0000000000001,-555.,113.));
#142834=CARTESIAN_POINT('Origin',(-115.,-555.,113.));
#142835=CARTESIAN_POINT('Origin',(90.,-555.,113.));
#142836=CARTESIAN_POINT('Origin',(-113.,-555.,115.));
#142837=CARTESIAN_POINT('Origin',(-113.,-555.,-90.));
#142838=CARTESIAN_POINT('Origin',(90.,-555.,90.));
#142839=CARTESIAN_POINT('Origin',(113.,-555.,90.));
#142840=CARTESIAN_POINT('Origin',(-90.0000000000001,-555.,-90.));
#142841=CARTESIAN_POINT('Origin',(-90.0000000000001,-555.,-113.));
#142842=CARTESIAN_POINT('Origin',(113.,-555.,115.));
#142843=CARTESIAN_POINT('Origin',(113.,-555.,-90.));
#142844=CARTESIAN_POINT('Origin',(-115.,-555.,-113.));
#142845=CARTESIAN_POINT('Origin',(90.,-555.,-113.));
#142846=CARTESIAN_POINT('Origin',(90.,-555.,-90.));
#276448=UNCERTAINTY_MEASURE_WITH_UNIT(LENGTH_MEASURE(0.01),#276463,
'DISTANCE_ACCURACY_VALUE',
'Maximum model space distance between geometric entities at asserted c
onnectivities');
#276454=UNCERTAINTY_MEASURE_WITH_UNIT(LENGTH_MEASURE(0.01),#276463,
'DISTANCE_ACCURACY_VALUE',
'Maximum model space distance between geometric entities at asserted c
onnectivities');
#276456=(
GEOMETRIC_REPRESENTATION_CONTEXT(3)
GLOBAL_UNCERTAINTY_ASSIGNED_CONTEXT((#276448))
GLOBAL_UNIT_ASSIGNED_CONTEXT((#276463,#276465,#276466))
REPRESENTATION_CONTEXT('','3D')
);
#276462=(
GEOMETRIC_REPRESENTATION_CONTEXT(3)
GLOBAL_UNCERTAINTY_ASSIGNED_CONTEXT((#276454))
GLOBAL_UNIT_ASSIGNED_CONTEXT((#276463,#276465,#276466))
REPRESENTATION_CONTEXT('','3D')
);
#276463=(
LENGTH_UNIT()
NAMED_UNIT(*)
SI_UNIT(.MILLI.,.METRE.)
);
#276465=(
NAMED_UNIT(*)
PLANE_ANGLE_UNIT()
SI_UNIT($,.RADIAN.)
);
#276466=(
NAMED_UNIT(*)
SI_UNIT($,.STERADIAN.)
SOLID_ANGLE_UNIT()
);
#276468=SHAPE_DEFINITION_REPRESENTATION(#276475,#276488);
#276475=PRODUCT_DEFINITION_SHAPE('',$,#276496);
#276488=SHAPE_REPRESENTATION('',(#98803),#276456);
#276494=PRODUCT_DEFINITION_CONTEXT('part definition',#276517,'design');
#276496=PRODUCT_DEFINITION('Stainless Steel Hopper Funnel',
'Stainless Steel Hopper Funnel',#276503,#276494);
#276503=PRODUCT_DEFINITION_FORMATION('',$,#276520);
#276517=APPLICATION_CONTEXT(
'Core Data for Automotive Mechanical Design Process');
#276518=PRODUCT_CONTEXT('part definition',#276517,'mechanical');
#276520=PRODUCT('Stainless Steel Hopper Funnel',
'Stainless Steel Hopper Funnel',$,(#276518));
#276527=PRESENTATION_STYLE_ASSIGNMENT((#276532));
#276532=SURFACE_STYLE_USAGE(.BOTH.,#276537);
#276537=SURFACE_SIDE_STYLE('',(#276542));
#276542=SURFACE_STYLE_FILL_AREA(#276547);
#276547=FILL_AREA_STYLE('Opaque(97,158,199)',(#276552));
#276552=FILL_AREA_STYLE_COLOUR('Opaque(97,158,199)',#276557);
#276557=COLOUR_RGB('Opaque(97,158,199)',0.380392156862745,0.619607843137255,
0.780392156862745);
ENDSEC;
END-ISO-10303-21;
